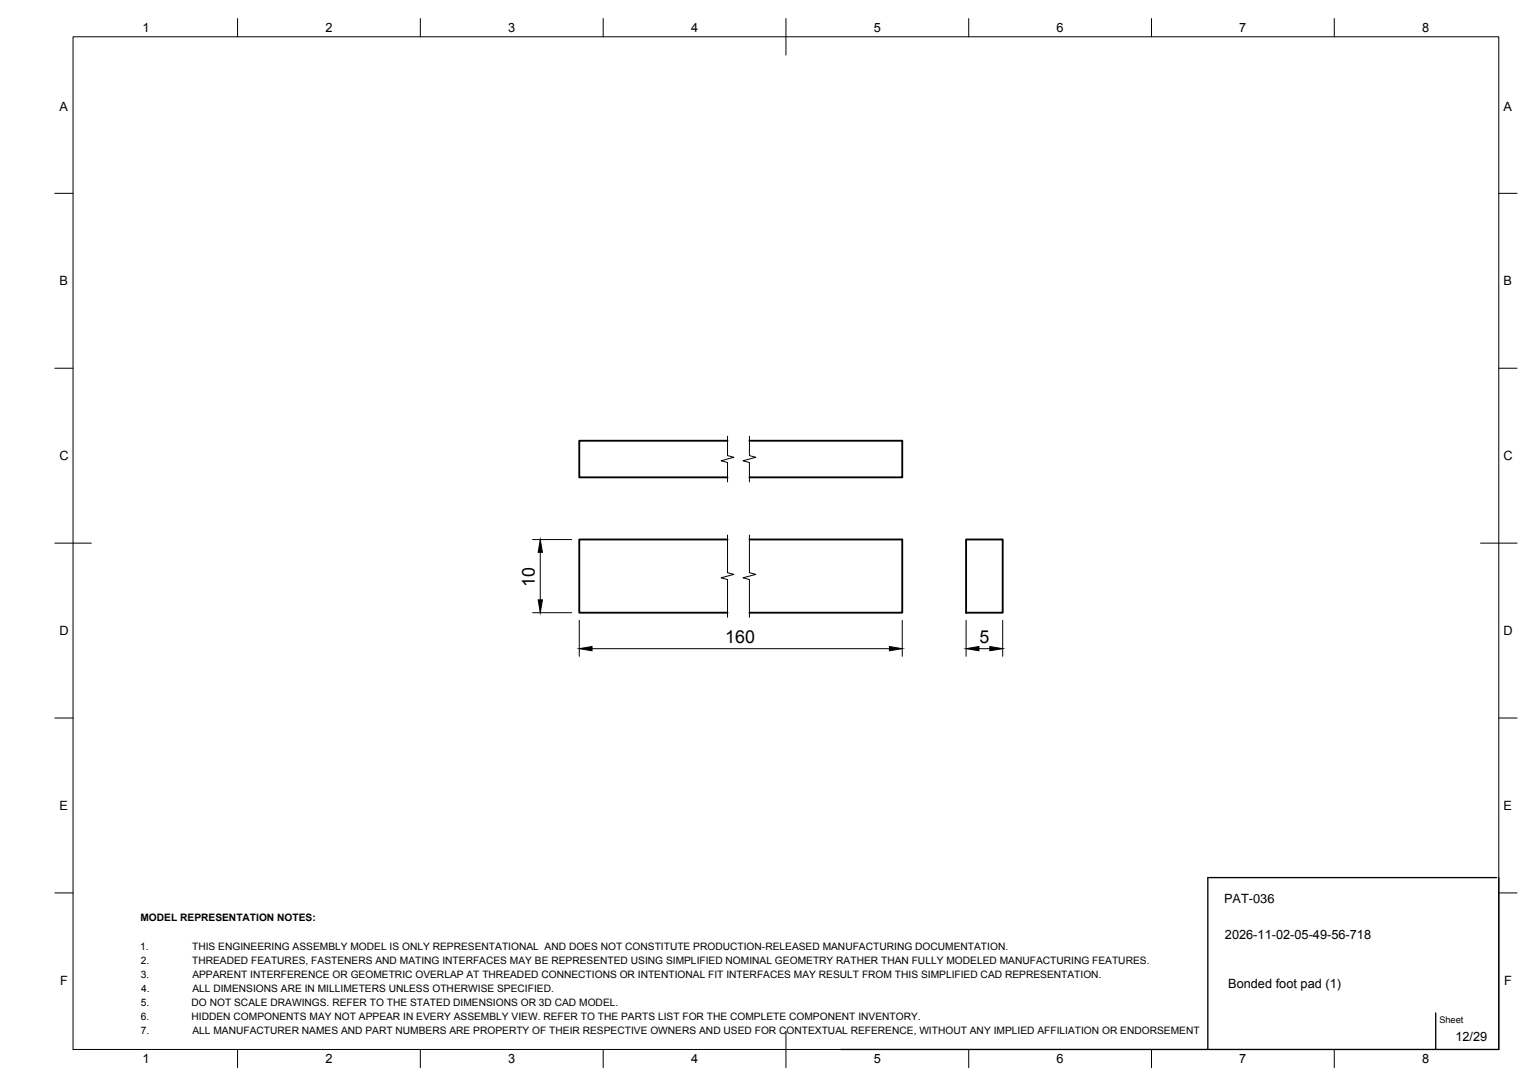
ISO-10303-21;
HEADER;
/* Generated by software containing ST-Developer
 * from STEP Tools, Inc. (www.steptools.com) 
 */

FILE_DESCRIPTION(
/* description */ ('Flange-mounted spindle'),
/* implementation_level */ '2;1');

FILE_NAME(
/* name */ 'Bonded foot pad (1).step',
/* time_stamp */ '2026-10-27T10:49:51-07:00',
/* author */ (''),
/* organization */ (''),
/* preprocessor_version */ 'ST-DEVELOPER v20.2',
/* originating_system */ 'Autodesk Translation Framework v15.17.0.0',
/* authorisation */ '');

FILE_SCHEMA (('AUTOMOTIVE_DESIGN { 1 0 10303 214 3 1 1 }'));
ENDSEC;

DATA;
#10=MECHANICAL_DESIGN_GEOMETRIC_PRESENTATION_REPRESENTATION('',(#345),#11764);
#291=SHAPE_REPRESENTATION_RELATIONSHIP('SRR','None',#11887,#318);
#318=ADVANCED_BREP_SHAPE_REPRESENTATION('',(#373),#11742);
#345=STYLED_ITEM('',(#12092),#373);
#373=MANIFOLD_SOLID_BREP('Body1',#6137);
#534=PLANE('',#6548);
#535=PLANE('',#6549);
#536=PLANE('',#6550);
#537=PLANE('',#6551);
#538=PLANE('',#6552);
#539=PLANE('',#6553);
#719=FACE_OUTER_BOUND('',#1090,.T.);
#720=FACE_OUTER_BOUND('',#1091,.T.);
#721=FACE_OUTER_BOUND('',#1092,.T.);
#722=FACE_OUTER_BOUND('',#1093,.T.);
#723=FACE_OUTER_BOUND('',#1094,.T.);
#724=FACE_OUTER_BOUND('',#1095,.T.);
#1090=EDGE_LOOP('',(#4191,#4192,#4193,#4194));
#1091=EDGE_LOOP('',(#4195,#4196,#4197,#4198));
#1092=EDGE_LOOP('',(#4199,#4200,#4201,#4202));
#1093=EDGE_LOOP('',(#4203,#4204,#4205,#4206));
#1094=EDGE_LOOP('',(#4207,#4208,#4209,#4210));
#1095=EDGE_LOOP('',(#4211,#4212,#4213,#4214));
#1538=LINE('',#9341,#1960);
#1539=LINE('',#9343,#1961);
#1540=LINE('',#9345,#1962);
#1541=LINE('',#9346,#1963);
#1542=LINE('',#9349,#1964);
#1543=LINE('',#9351,#1965);
#1544=LINE('',#9352,#1966);
#1545=LINE('',#9355,#1967);
#1546=LINE('',#9357,#1968);
#1547=LINE('',#9358,#1969);
#1548=LINE('',#9360,#1970);
#1549=LINE('',#9361,#1971);
#1960=VECTOR('',#7447,1.);
#1961=VECTOR('',#7448,1.);
#1962=VECTOR('',#7449,1.);
#1963=VECTOR('',#7450,1.);
#1964=VECTOR('',#7453,1.);
#1965=VECTOR('',#7454,1.);
#1966=VECTOR('',#7455,1.);
#1967=VECTOR('',#7458,1.);
#1968=VECTOR('',#7459,1.);
#1969=VECTOR('',#7460,1.);
#1970=VECTOR('',#7463,1.);
#1971=VECTOR('',#7464,1.);
#2711=VERTEX_POINT('',#9339);
#2712=VERTEX_POINT('',#9340);
#2713=VERTEX_POINT('',#9342);
#2714=VERTEX_POINT('',#9344);
#2715=VERTEX_POINT('',#9348);
#2716=VERTEX_POINT('',#9350);
#2717=VERTEX_POINT('',#9354);
#2718=VERTEX_POINT('',#9356);
#3288=EDGE_CURVE('',#2711,#2712,#1538,.T.);
#3289=EDGE_CURVE('',#2712,#2713,#1539,.T.);
#3290=EDGE_CURVE('',#2714,#2713,#1540,.T.);
#3291=EDGE_CURVE('',#2711,#2714,#1541,.T.);
#3292=EDGE_CURVE('',#2715,#2711,#1542,.T.);
#3293=EDGE_CURVE('',#2716,#2714,#1543,.T.);
#3294=EDGE_CURVE('',#2715,#2716,#1544,.T.);
#3295=EDGE_CURVE('',#2717,#2715,#1545,.T.);
#3296=EDGE_CURVE('',#2718,#2716,#1546,.T.);
#3297=EDGE_CURVE('',#2717,#2718,#1547,.T.);
#3298=EDGE_CURVE('',#2712,#2717,#1548,.T.);
#3299=EDGE_CURVE('',#2713,#2718,#1549,.T.);
#4191=ORIENTED_EDGE('',*,*,#3288,.T.);
#4192=ORIENTED_EDGE('',*,*,#3289,.T.);
#4193=ORIENTED_EDGE('',*,*,#3290,.F.);
#4194=ORIENTED_EDGE('',*,*,#3291,.F.);
#4195=ORIENTED_EDGE('',*,*,#3292,.T.);
#4196=ORIENTED_EDGE('',*,*,#3291,.T.);
#4197=ORIENTED_EDGE('',*,*,#3293,.F.);
#4198=ORIENTED_EDGE('',*,*,#3294,.F.);
#4199=ORIENTED_EDGE('',*,*,#3295,.T.);
#4200=ORIENTED_EDGE('',*,*,#3294,.T.);
#4201=ORIENTED_EDGE('',*,*,#3296,.F.);
#4202=ORIENTED_EDGE('',*,*,#3297,.F.);
#4203=ORIENTED_EDGE('',*,*,#3298,.T.);
#4204=ORIENTED_EDGE('',*,*,#3297,.T.);
#4205=ORIENTED_EDGE('',*,*,#3299,.F.);
#4206=ORIENTED_EDGE('',*,*,#3289,.F.);
#4207=ORIENTED_EDGE('',*,*,#3299,.T.);
#4208=ORIENTED_EDGE('',*,*,#3296,.T.);
#4209=ORIENTED_EDGE('',*,*,#3293,.T.);
#4210=ORIENTED_EDGE('',*,*,#3290,.T.);
#4211=ORIENTED_EDGE('',*,*,#3298,.F.);
#4212=ORIENTED_EDGE('',*,*,#3288,.F.);
#4213=ORIENTED_EDGE('',*,*,#3292,.F.);
#4214=ORIENTED_EDGE('',*,*,#3295,.F.);
#5830=ADVANCED_FACE('',(#719),#534,.T.);
#5831=ADVANCED_FACE('',(#720),#535,.T.);
#5832=ADVANCED_FACE('',(#721),#536,.T.);
#5833=ADVANCED_FACE('',(#722),#537,.T.);
#5834=ADVANCED_FACE('',(#723),#538,.T.);
#5835=ADVANCED_FACE('',(#724),#539,.F.);
#6137=CLOSED_SHELL('',(#5830,#5831,#5832,#5833,#5834,#5835));
#6547=AXIS2_PLACEMENT_3D('',#9337,#7443,#7444);
#6548=AXIS2_PLACEMENT_3D('',#9338,#7445,#7446);
#6549=AXIS2_PLACEMENT_3D('',#9347,#7451,#7452);
#6550=AXIS2_PLACEMENT_3D('',#9353,#7456,#7457);
#6551=AXIS2_PLACEMENT_3D('',#9359,#7461,#7462);
#6552=AXIS2_PLACEMENT_3D('',#9362,#7465,#7466);
#6553=AXIS2_PLACEMENT_3D('',#9363,#7467,#7468);
#7443=DIRECTION('axis',(0.,0.,1.));
#7444=DIRECTION('refdir',(1.,0.,0.));
#7445=DIRECTION('center_axis',(0.,1.,0.));
#7446=DIRECTION('ref_axis',(-1.,0.,0.));
#7447=DIRECTION('',(-1.,0.,0.));
#7448=DIRECTION('',(0.,0.,1.));
#7449=DIRECTION('',(-1.,0.,0.));
#7450=DIRECTION('',(0.,0.,1.));
#7451=DIRECTION('center_axis',(1.,0.,0.));
#7452=DIRECTION('ref_axis',(0.,1.,0.));
#7453=DIRECTION('',(0.,1.,0.));
#7454=DIRECTION('',(0.,1.,0.));
#7455=DIRECTION('',(0.,0.,1.));
#7456=DIRECTION('center_axis',(0.,-1.,0.));
#7457=DIRECTION('ref_axis',(1.,0.,0.));
#7458=DIRECTION('',(1.,0.,0.));
#7459=DIRECTION('',(1.,0.,0.));
#7460=DIRECTION('',(0.,0.,1.));
#7461=DIRECTION('center_axis',(-1.,0.,0.));
#7462=DIRECTION('ref_axis',(0.,-1.,0.));
#7463=DIRECTION('',(0.,-1.,0.));
#7464=DIRECTION('',(0.,-1.,0.));
#7465=DIRECTION('center_axis',(0.,0.,1.));
#7466=DIRECTION('ref_axis',(1.,0.,0.));
#7467=DIRECTION('center_axis',(0.,0.,1.));
#7468=DIRECTION('ref_axis',(1.,0.,0.));
#9337=CARTESIAN_POINT('',(0.,0.,0.));
#9338=CARTESIAN_POINT('Origin',(8.,4.,-0.5));
#9339=CARTESIAN_POINT('',(8.,4.,-0.5));
#9340=CARTESIAN_POINT('',(-8.,4.,-0.5));
#9341=CARTESIAN_POINT('',(8.,4.,-0.5));
#9342=CARTESIAN_POINT('',(-8.,4.,0.));
#9343=CARTESIAN_POINT('',(-8.,4.,-0.5));
#9344=CARTESIAN_POINT('',(8.,4.,0.));
#9345=CARTESIAN_POINT('',(8.,4.,0.));
#9346=CARTESIAN_POINT('',(8.,4.,-0.5));
#9347=CARTESIAN_POINT('Origin',(8.,3.,-0.5));
#9348=CARTESIAN_POINT('',(8.,3.,-0.5));
#9349=CARTESIAN_POINT('',(8.,3.,-0.5));
#9350=CARTESIAN_POINT('',(8.,3.,0.));
#9351=CARTESIAN_POINT('',(8.,3.,0.));
#9352=CARTESIAN_POINT('',(8.,3.,-0.5));
#9353=CARTESIAN_POINT('Origin',(-8.,3.,-0.5));
#9354=CARTESIAN_POINT('',(-8.,3.,-0.5));
#9355=CARTESIAN_POINT('',(-8.,3.,-0.5));
#9356=CARTESIAN_POINT('',(-8.,3.,0.));
#9357=CARTESIAN_POINT('',(-8.,3.,0.));
#9358=CARTESIAN_POINT('',(-8.,3.,-0.5));
#9359=CARTESIAN_POINT('Origin',(-8.,4.,-0.5));
#9360=CARTESIAN_POINT('',(-8.,4.,-0.5));
#9361=CARTESIAN_POINT('',(-8.,4.,0.));
#9362=CARTESIAN_POINT('Origin',(0.,3.5,0.));
#9363=CARTESIAN_POINT('Origin',(0.,3.5,-0.5));
#11710=UNCERTAINTY_MEASURE_WITH_UNIT(LENGTH_MEASURE(0.001),#11765,
'DISTANCE_ACCURACY_VALUE',
'Maximum model space distance between geometric entities at asserted c
onnectivities');
#11732=UNCERTAINTY_MEASURE_WITH_UNIT(LENGTH_MEASURE(0.001),#11765,
'DISTANCE_ACCURACY_VALUE',
'Maximum model space distance between geometric entities at asserted c
onnectivities');
#11742=(
GEOMETRIC_REPRESENTATION_CONTEXT(3)
GLOBAL_UNCERTAINTY_ASSIGNED_CONTEXT((#11710))
GLOBAL_UNIT_ASSIGNED_CONTEXT((#11765,#11767,#11768))
REPRESENTATION_CONTEXT('','3D')
);
#11764=(
GEOMETRIC_REPRESENTATION_CONTEXT(3)
GLOBAL_UNCERTAINTY_ASSIGNED_CONTEXT((#11732))
GLOBAL_UNIT_ASSIGNED_CONTEXT((#11765,#11767,#11768))
REPRESENTATION_CONTEXT('','3D')
);
#11765=(
LENGTH_UNIT()
NAMED_UNIT(*)
SI_UNIT(.CENTI.,.METRE.)
);
#11767=(
NAMED_UNIT(*)
PLANE_ANGLE_UNIT()
SI_UNIT($,.RADIAN.)
);
#11768=(
NAMED_UNIT(*)
SI_UNIT($,.STERADIAN.)
SOLID_ANGLE_UNIT()
);
#11778=SHAPE_DEFINITION_REPRESENTATION(#11809,#11887);
#11809=PRODUCT_DEFINITION_SHAPE('',$,#11919);
#11887=SHAPE_REPRESENTATION('',(#6547),#11742);
#11909=PRODUCT_DEFINITION_CONTEXT('part definition',#12004,'design');
#11919=PRODUCT_DEFINITION('Bonded foot pad (1)','Bonded foot pad (1)',#11950,
#11909);
#11950=PRODUCT_DEFINITION_FORMATION('',$,#12015);
#12004=APPLICATION_CONTEXT(
'Core Data for Automotive Mechanical Design Process');
#12005=PRODUCT_CONTEXT('part definition',#12004,'mechanical');
#12015=PRODUCT('Bonded foot pad (1)','Bonded foot pad (1)',
'Bonded foot pad (1)',(#12005));
#12086=COLOUR_RGB('Sky Blue',0.24,0.69,0.87);
#12087=FILL_AREA_STYLE_COLOUR('',#12086);
#12088=FILL_AREA_STYLE('',(#12087));
#12089=SURFACE_STYLE_FILL_AREA(#12088);
#12090=SURFACE_SIDE_STYLE('',(#12089));
#12091=SURFACE_STYLE_USAGE(.BOTH.,#12090);
#12092=PRESENTATION_STYLE_ASSIGNMENT((#12091));
ENDSEC;
END-ISO-10303-21;
